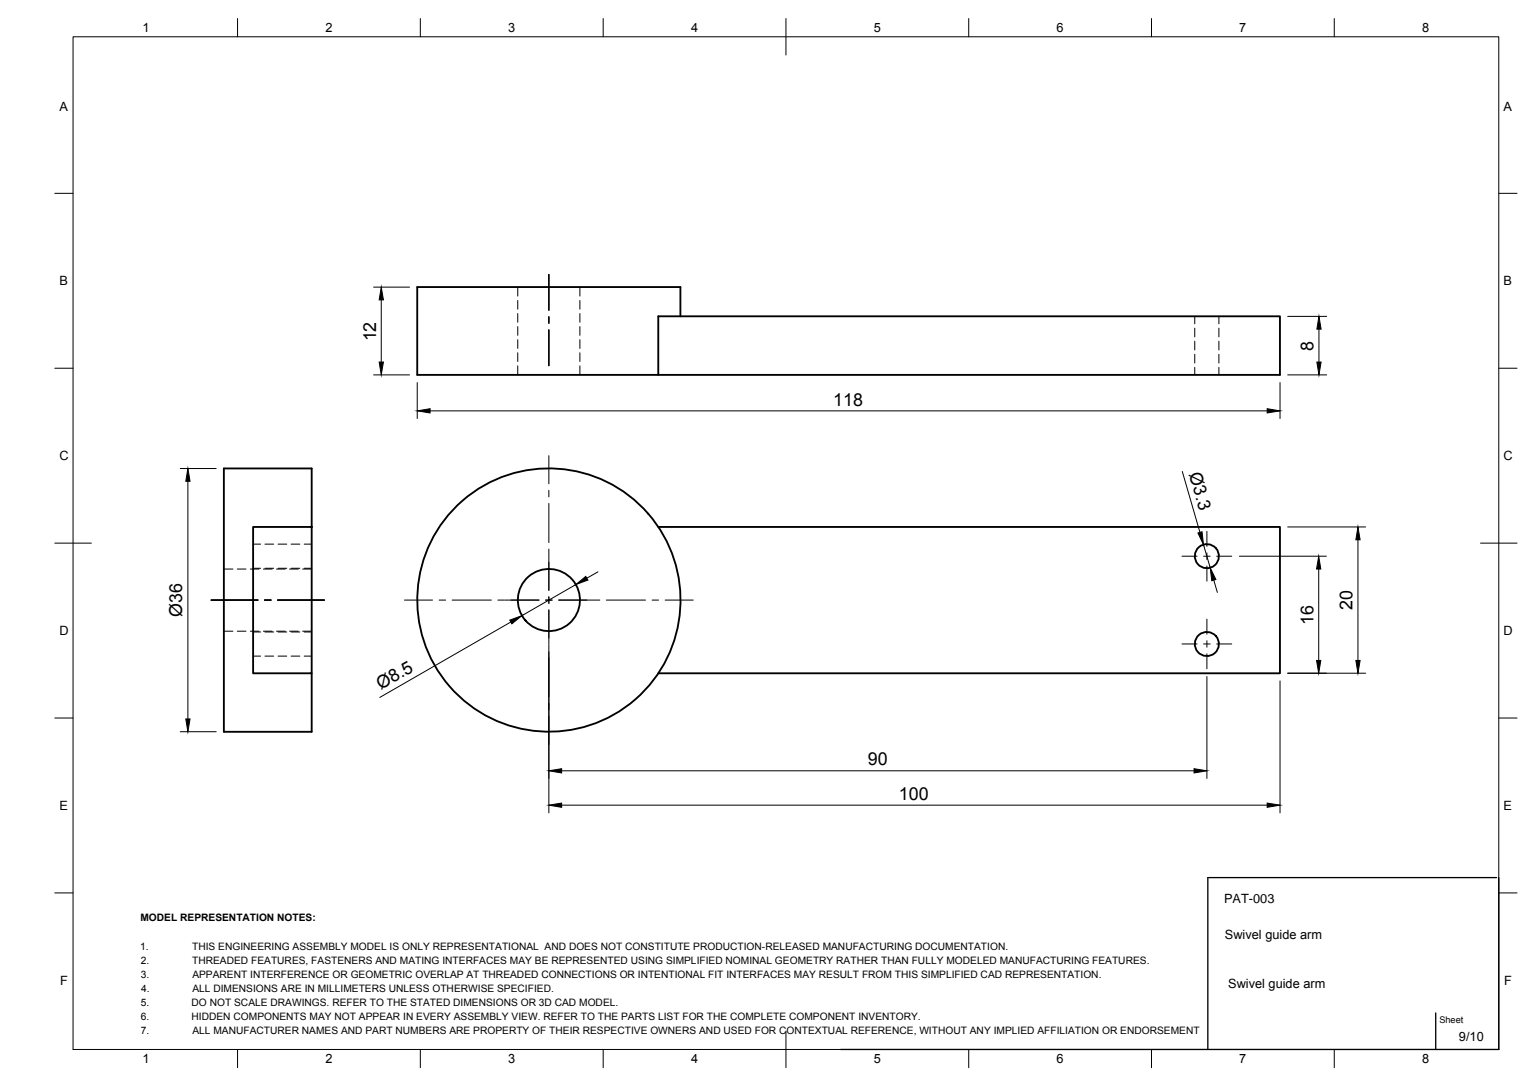
ISO-10303-21;
HEADER;
/* Generated by software containing ST-Developer
 * from STEP Tools, Inc. (www.steptools.com) 
 */

FILE_DESCRIPTION(
/* description */ ('PAT-003'),
/* implementation_level */ '2;1');

FILE_NAME(
/* name */ 'Swivel guide arm.step',
/* time_stamp */ '2026-10-29T15:45:40-07:00',
/* author */ (''),
/* organization */ (''),
/* preprocessor_version */ 'ST-DEVELOPER v20.2',
/* originating_system */ 'Autodesk Translation Framework v15.17.0.0',
/* authorisation */ '');

FILE_SCHEMA (('AUTOMOTIVE_DESIGN { 1 0 10303 214 3 1 1 }'));
ENDSEC;

DATA;
#10=MECHANICAL_DESIGN_GEOMETRIC_PRESENTATION_REPRESENTATION('',(#153),#5761);
#129=SHAPE_REPRESENTATION_RELATIONSHIP('SRR','None',#5824,#141);
#141=ADVANCED_BREP_SHAPE_REPRESENTATION('',(#164),#5755);
#153=STYLED_ITEM('',(#5942),#164);
#164=MANIFOLD_SOLID_BREP('Body1',#3328);
#186=FACE_BOUND('',#659,.T.);
#187=FACE_BOUND('',#660,.T.);
#188=FACE_BOUND('',#661,.T.);
#189=FACE_BOUND('',#666,.T.);
#190=FACE_BOUND('',#667,.T.);
#191=FACE_BOUND('',#671,.T.);
#297=PLANE('',#3633);
#298=PLANE('',#3637);
#299=PLANE('',#3638);
#300=PLANE('',#3639);
#301=PLANE('',#3640);
#302=PLANE('',#3646);
#452=FACE_OUTER_BOUND('',#656,.T.);
#453=FACE_OUTER_BOUND('',#657,.T.);
#454=FACE_OUTER_BOUND('',#658,.T.);
#455=FACE_OUTER_BOUND('',#662,.T.);
#456=FACE_OUTER_BOUND('',#663,.T.);
#457=FACE_OUTER_BOUND('',#664,.T.);
#458=FACE_OUTER_BOUND('',#665,.T.);
#459=FACE_OUTER_BOUND('',#668,.T.);
#460=FACE_OUTER_BOUND('',#669,.T.);
#461=FACE_OUTER_BOUND('',#670,.T.);
#656=EDGE_LOOP('',(#2758,#2759,#2760,#2761));
#657=EDGE_LOOP('',(#2762,#2763,#2764,#2765));
#658=EDGE_LOOP('',(#2766,#2767,#2768,#2769,#2770));
#659=EDGE_LOOP('',(#2771));
#660=EDGE_LOOP('',(#2772));
#661=EDGE_LOOP('',(#2773));
#662=EDGE_LOOP('',(#2774,#2775,#2776,#2777));
#663=EDGE_LOOP('',(#2778,#2779,#2780,#2781));
#664=EDGE_LOOP('',(#2782,#2783,#2784,#2785));
#665=EDGE_LOOP('',(#2786,#2787,#2788,#2789));
#666=EDGE_LOOP('',(#2790));
#667=EDGE_LOOP('',(#2791));
#668=EDGE_LOOP('',(#2792,#2793,#2794,#2795,#2796,#2797,#2798,#2799));
#669=EDGE_LOOP('',(#2800,#2801,#2802,#2803));
#670=EDGE_LOOP('',(#2804));
#671=EDGE_LOOP('',(#2805));
#978=LINE('',#5332,#1300);
#979=LINE('',#5338,#1301);
#980=LINE('',#5347,#1302);
#981=LINE('',#5349,#1303);
#982=LINE('',#5350,#1304);
#983=LINE('',#5355,#1305);
#984=LINE('',#5357,#1306);
#985=LINE('',#5358,#1307);
#986=LINE('',#5361,#1308);
#987=LINE('',#5362,#1309);
#988=LINE('',#5365,#1310);
#989=LINE('',#5366,#1311);
#990=LINE('',#5371,#1312);
#991=LINE('',#5375,#1313);
#1300=VECTOR('',#4335,0.164999999999999);
#1301=VECTOR('',#4342,0.164999999999999);
#1302=VECTOR('',#4351,1.);
#1303=VECTOR('',#4352,1.);
#1304=VECTOR('',#4353,1.);
#1305=VECTOR('',#4358,1.);
#1306=VECTOR('',#4359,1.);
#1307=VECTOR('',#4360,1.);
#1308=VECTOR('',#4363,1.);
#1309=VECTOR('',#4364,1.);
#1310=VECTOR('',#4367,1.);
#1311=VECTOR('',#4368,1.);
#1312=VECTOR('',#4375,1.8);
#1313=VECTOR('',#4380,0.425);
#1432=CIRCLE('',#3628,0.164999999999999);
#1433=CIRCLE('',#3629,0.164999999999999);
#1434=CIRCLE('',#3631,0.164999999999999);
#1435=CIRCLE('',#3632,0.164999999999999);
#1436=CIRCLE('',#3634,1.8);
#1437=CIRCLE('',#3635,1.8);
#1438=CIRCLE('',#3636,0.425);
#1439=CIRCLE('',#3641,1.8);
#1440=CIRCLE('',#3643,1.8);
#1441=CIRCLE('',#3645,0.425);
#1670=VERTEX_POINT('',#5329);
#1671=VERTEX_POINT('',#5331);
#1672=VERTEX_POINT('',#5335);
#1673=VERTEX_POINT('',#5337);
#1674=VERTEX_POINT('',#5341);
#1675=VERTEX_POINT('',#5342);
#1676=VERTEX_POINT('',#5344);
#1677=VERTEX_POINT('',#5346);
#1678=VERTEX_POINT('',#5348);
#1679=VERTEX_POINT('',#5351);
#1680=VERTEX_POINT('',#5354);
#1681=VERTEX_POINT('',#5356);
#1682=VERTEX_POINT('',#5360);
#1683=VERTEX_POINT('',#5364);
#1684=VERTEX_POINT('',#5370);
#1685=VERTEX_POINT('',#5374);
#2050=EDGE_CURVE('',#1670,#1670,#1432,.T.);
#2051=EDGE_CURVE('',#1670,#1671,#978,.T.);
#2052=EDGE_CURVE('',#1671,#1671,#1433,.T.);
#2053=EDGE_CURVE('',#1672,#1672,#1434,.T.);
#2054=EDGE_CURVE('',#1672,#1673,#979,.T.);
#2055=EDGE_CURVE('',#1673,#1673,#1435,.T.);
#2056=EDGE_CURVE('',#1674,#1675,#1436,.T.);
#2057=EDGE_CURVE('',#1675,#1676,#1437,.T.);
#2058=EDGE_CURVE('',#1676,#1677,#980,.T.);
#2059=EDGE_CURVE('',#1677,#1678,#981,.T.);
#2060=EDGE_CURVE('',#1678,#1674,#982,.T.);
#2061=EDGE_CURVE('',#1679,#1679,#1438,.T.);
#2062=EDGE_CURVE('',#1674,#1680,#983,.T.);
#2063=EDGE_CURVE('',#1681,#1678,#984,.T.);
#2064=EDGE_CURVE('',#1681,#1680,#985,.T.);
#2065=EDGE_CURVE('',#1682,#1681,#986,.T.);
#2066=EDGE_CURVE('',#1682,#1677,#987,.T.);
#2067=EDGE_CURVE('',#1683,#1676,#988,.T.);
#2068=EDGE_CURVE('',#1683,#1682,#989,.T.);
#2069=EDGE_CURVE('',#1680,#1683,#1439,.T.);
#2070=EDGE_CURVE('',#1675,#1684,#990,.T.);
#2071=EDGE_CURVE('',#1684,#1684,#1440,.T.);
#2072=EDGE_CURVE('',#1679,#1685,#991,.T.);
#2073=EDGE_CURVE('',#1685,#1685,#1441,.T.);
#2758=ORIENTED_EDGE('',*,*,#2050,.F.);
#2759=ORIENTED_EDGE('',*,*,#2051,.T.);
#2760=ORIENTED_EDGE('',*,*,#2052,.F.);
#2761=ORIENTED_EDGE('',*,*,#2051,.F.);
#2762=ORIENTED_EDGE('',*,*,#2053,.F.);
#2763=ORIENTED_EDGE('',*,*,#2054,.T.);
#2764=ORIENTED_EDGE('',*,*,#2055,.F.);
#2765=ORIENTED_EDGE('',*,*,#2054,.F.);
#2766=ORIENTED_EDGE('',*,*,#2056,.T.);
#2767=ORIENTED_EDGE('',*,*,#2057,.T.);
#2768=ORIENTED_EDGE('',*,*,#2058,.T.);
#2769=ORIENTED_EDGE('',*,*,#2059,.T.);
#2770=ORIENTED_EDGE('',*,*,#2060,.T.);
#2771=ORIENTED_EDGE('',*,*,#2052,.T.);
#2772=ORIENTED_EDGE('',*,*,#2055,.T.);
#2773=ORIENTED_EDGE('',*,*,#2061,.T.);
#2774=ORIENTED_EDGE('',*,*,#2062,.F.);
#2775=ORIENTED_EDGE('',*,*,#2060,.F.);
#2776=ORIENTED_EDGE('',*,*,#2063,.F.);
#2777=ORIENTED_EDGE('',*,*,#2064,.T.);
#2778=ORIENTED_EDGE('',*,*,#2065,.T.);
#2779=ORIENTED_EDGE('',*,*,#2063,.T.);
#2780=ORIENTED_EDGE('',*,*,#2059,.F.);
#2781=ORIENTED_EDGE('',*,*,#2066,.F.);
#2782=ORIENTED_EDGE('',*,*,#2067,.F.);
#2783=ORIENTED_EDGE('',*,*,#2068,.T.);
#2784=ORIENTED_EDGE('',*,*,#2066,.T.);
#2785=ORIENTED_EDGE('',*,*,#2058,.F.);
#2786=ORIENTED_EDGE('',*,*,#2069,.F.);
#2787=ORIENTED_EDGE('',*,*,#2064,.F.);
#2788=ORIENTED_EDGE('',*,*,#2065,.F.);
#2789=ORIENTED_EDGE('',*,*,#2068,.F.);
#2790=ORIENTED_EDGE('',*,*,#2050,.T.);
#2791=ORIENTED_EDGE('',*,*,#2053,.T.);
#2792=ORIENTED_EDGE('',*,*,#2062,.T.);
#2793=ORIENTED_EDGE('',*,*,#2069,.T.);
#2794=ORIENTED_EDGE('',*,*,#2067,.T.);
#2795=ORIENTED_EDGE('',*,*,#2057,.F.);
#2796=ORIENTED_EDGE('',*,*,#2070,.T.);
#2797=ORIENTED_EDGE('',*,*,#2071,.T.);
#2798=ORIENTED_EDGE('',*,*,#2070,.F.);
#2799=ORIENTED_EDGE('',*,*,#2056,.F.);
#2800=ORIENTED_EDGE('',*,*,#2061,.F.);
#2801=ORIENTED_EDGE('',*,*,#2072,.T.);
#2802=ORIENTED_EDGE('',*,*,#2073,.T.);
#2803=ORIENTED_EDGE('',*,*,#2072,.F.);
#2804=ORIENTED_EDGE('',*,*,#2071,.F.);
#2805=ORIENTED_EDGE('',*,*,#2073,.F.);
#3108=CYLINDRICAL_SURFACE('',#3627,0.164999999999999);
#3109=CYLINDRICAL_SURFACE('',#3630,0.164999999999999);
#3110=CYLINDRICAL_SURFACE('',#3642,1.8);
#3111=CYLINDRICAL_SURFACE('',#3644,0.425);
#3245=ADVANCED_FACE('',(#452),#3108,.F.);
#3246=ADVANCED_FACE('',(#453),#3109,.F.);
#3247=ADVANCED_FACE('',(#454,#186,#187,#188),#297,.T.);
#3248=ADVANCED_FACE('',(#455),#298,.T.);
#3249=ADVANCED_FACE('',(#456),#299,.T.);
#3250=ADVANCED_FACE('',(#457),#300,.T.);
#3251=ADVANCED_FACE('',(#458,#189,#190),#301,.F.);
#3252=ADVANCED_FACE('',(#459),#3110,.T.);
#3253=ADVANCED_FACE('',(#460),#3111,.F.);
#3254=ADVANCED_FACE('',(#461,#191),#302,.F.);
#3328=CLOSED_SHELL('',(#3245,#3246,#3247,#3248,#3249,#3250,#3251,#3252,
#3253,#3254));
#3626=AXIS2_PLACEMENT_3D('',#5327,#4329,#4330);
#3627=AXIS2_PLACEMENT_3D('',#5328,#4331,#4332);
#3628=AXIS2_PLACEMENT_3D('',#5330,#4333,#4334);
#3629=AXIS2_PLACEMENT_3D('',#5333,#4336,#4337);
#3630=AXIS2_PLACEMENT_3D('',#5334,#4338,#4339);
#3631=AXIS2_PLACEMENT_3D('',#5336,#4340,#4341);
#3632=AXIS2_PLACEMENT_3D('',#5339,#4343,#4344);
#3633=AXIS2_PLACEMENT_3D('',#5340,#4345,#4346);
#3634=AXIS2_PLACEMENT_3D('',#5343,#4347,#4348);
#3635=AXIS2_PLACEMENT_3D('',#5345,#4349,#4350);
#3636=AXIS2_PLACEMENT_3D('',#5352,#4354,#4355);
#3637=AXIS2_PLACEMENT_3D('',#5353,#4356,#4357);
#3638=AXIS2_PLACEMENT_3D('',#5359,#4361,#4362);
#3639=AXIS2_PLACEMENT_3D('',#5363,#4365,#4366);
#3640=AXIS2_PLACEMENT_3D('',#5367,#4369,#4370);
#3641=AXIS2_PLACEMENT_3D('',#5368,#4371,#4372);
#3642=AXIS2_PLACEMENT_3D('',#5369,#4373,#4374);
#3643=AXIS2_PLACEMENT_3D('',#5372,#4376,#4377);
#3644=AXIS2_PLACEMENT_3D('',#5373,#4378,#4379);
#3645=AXIS2_PLACEMENT_3D('',#5376,#4381,#4382);
#3646=AXIS2_PLACEMENT_3D('',#5377,#4383,#4384);
#4329=DIRECTION('axis',(0.,0.,1.));
#4330=DIRECTION('refdir',(1.,0.,0.));
#4331=DIRECTION('center_axis',(0.,0.,1.));
#4332=DIRECTION('ref_axis',(1.,0.,0.));
#4333=DIRECTION('center_axis',(0.,0.,1.));
#4334=DIRECTION('ref_axis',(1.,0.,0.));
#4335=DIRECTION('',(0.,0.,1.));
#4336=DIRECTION('center_axis',(0.,0.,-1.));
#4337=DIRECTION('ref_axis',(1.,0.,0.));
#4338=DIRECTION('center_axis',(0.,0.,1.));
#4339=DIRECTION('ref_axis',(1.,0.,0.));
#4340=DIRECTION('center_axis',(0.,0.,1.));
#4341=DIRECTION('ref_axis',(1.,0.,0.));
#4342=DIRECTION('',(0.,0.,1.));
#4343=DIRECTION('center_axis',(0.,0.,-1.));
#4344=DIRECTION('ref_axis',(1.,0.,0.));
#4345=DIRECTION('center_axis',(0.,0.,1.));
#4346=DIRECTION('ref_axis',(1.,0.,0.));
#4347=DIRECTION('center_axis',(0.,0.,1.));
#4348=DIRECTION('ref_axis',(1.,0.,0.));
#4349=DIRECTION('center_axis',(0.,0.,1.));
#4350=DIRECTION('ref_axis',(1.,0.,0.));
#4351=DIRECTION('',(1.,0.,0.));
#4352=DIRECTION('',(0.,1.,0.));
#4353=DIRECTION('',(-1.,0.,0.));
#4354=DIRECTION('center_axis',(0.,0.,-1.));
#4355=DIRECTION('ref_axis',(1.,0.,0.));
#4356=DIRECTION('center_axis',(0.,1.,0.));
#4357=DIRECTION('ref_axis',(-1.,0.,0.));
#4358=DIRECTION('',(0.,0.,-1.));
#4359=DIRECTION('',(0.,0.,1.));
#4360=DIRECTION('',(-1.,0.,0.));
#4361=DIRECTION('center_axis',(1.,0.,0.));
#4362=DIRECTION('ref_axis',(0.,1.,0.));
#4363=DIRECTION('',(0.,1.,0.));
#4364=DIRECTION('',(0.,0.,1.));
#4365=DIRECTION('center_axis',(0.,-1.,0.));
#4366=DIRECTION('ref_axis',(1.,0.,0.));
#4367=DIRECTION('',(0.,0.,1.));
#4368=DIRECTION('',(1.,0.,0.));
#4369=DIRECTION('center_axis',(0.,0.,1.));
#4370=DIRECTION('ref_axis',(1.,0.,0.));
#4371=DIRECTION('center_axis',(0.,0.,-1.));
#4372=DIRECTION('ref_axis',(1.,0.,0.));
#4373=DIRECTION('center_axis',(0.,0.,1.));
#4374=DIRECTION('ref_axis',(1.,0.,0.));
#4375=DIRECTION('',(0.,0.,-1.));
#4376=DIRECTION('center_axis',(0.,0.,1.));
#4377=DIRECTION('ref_axis',(1.,0.,0.));
#4378=DIRECTION('center_axis',(0.,0.,1.));
#4379=DIRECTION('ref_axis',(1.,0.,0.));
#4380=DIRECTION('',(0.,0.,-1.));
#4381=DIRECTION('center_axis',(0.,0.,-1.));
#4382=DIRECTION('ref_axis',(1.,0.,0.));
#4383=DIRECTION('center_axis',(0.,0.,1.));
#4384=DIRECTION('ref_axis',(1.,0.,0.));
#5327=CARTESIAN_POINT('',(0.,0.,0.));
#5328=CARTESIAN_POINT('Origin',(14.,-0.6,4.7));
#5329=CARTESIAN_POINT('',(13.835,-0.6,4.8));
#5330=CARTESIAN_POINT('Origin',(14.,-0.6,4.8));
#5331=CARTESIAN_POINT('',(13.835,-0.6,5.6));
#5332=CARTESIAN_POINT('',(13.835,-0.6,4.7));
#5333=CARTESIAN_POINT('Origin',(14.,-0.6,5.6));
#5334=CARTESIAN_POINT('Origin',(14.,0.6,4.7));
#5335=CARTESIAN_POINT('',(13.835,0.6,4.8));
#5336=CARTESIAN_POINT('Origin',(14.,0.6,4.8));
#5337=CARTESIAN_POINT('',(13.835,0.6,5.6));
#5338=CARTESIAN_POINT('',(13.835,0.6,4.7));
#5339=CARTESIAN_POINT('Origin',(14.,0.6,5.6));
#5340=CARTESIAN_POINT('Origin',(5.,0.,5.6));
#5341=CARTESIAN_POINT('',(6.49666295470958,1.,5.6));
#5342=CARTESIAN_POINT('',(3.2,-2.20436423846524E-16,5.6));
#5343=CARTESIAN_POINT('Origin',(5.,0.,5.6));
#5344=CARTESIAN_POINT('',(6.49666295470958,-1.,5.6));
#5345=CARTESIAN_POINT('Origin',(5.,0.,5.6));
#5346=CARTESIAN_POINT('',(15.,-1.,5.6));
#5347=CARTESIAN_POINT('',(5.,-1.,5.6));
#5348=CARTESIAN_POINT('',(15.,1.,5.6));
#5349=CARTESIAN_POINT('',(15.,-1.,5.6));
#5350=CARTESIAN_POINT('',(15.,1.,5.6));
#5351=CARTESIAN_POINT('',(4.575,-5.20474889637625E-17,5.6));
#5352=CARTESIAN_POINT('Origin',(5.,0.,5.6));
#5353=CARTESIAN_POINT('Origin',(15.,1.,4.8));
#5354=CARTESIAN_POINT('',(6.49666295470958,1.,4.8));
#5355=CARTESIAN_POINT('',(6.49666295470958,1.,4.4));
#5356=CARTESIAN_POINT('',(15.,1.,4.8));
#5357=CARTESIAN_POINT('',(15.,1.,4.8));
#5358=CARTESIAN_POINT('',(15.,1.,4.8));
#5359=CARTESIAN_POINT('Origin',(15.,-1.,4.8));
#5360=CARTESIAN_POINT('',(15.,-1.,4.8));
#5361=CARTESIAN_POINT('',(15.,-1.,4.8));
#5362=CARTESIAN_POINT('',(15.,-1.,4.8));
#5363=CARTESIAN_POINT('Origin',(5.,-1.,4.8));
#5364=CARTESIAN_POINT('',(6.49666295470958,-1.,4.8));
#5365=CARTESIAN_POINT('',(6.49666295470958,-1.,4.4));
#5366=CARTESIAN_POINT('',(5.,-1.,4.8));
#5367=CARTESIAN_POINT('Origin',(10.,0.,4.8));
#5368=CARTESIAN_POINT('Origin',(5.,0.,4.8));
#5369=CARTESIAN_POINT('Origin',(5.,0.,4.4));
#5370=CARTESIAN_POINT('',(3.2,-2.20436423846524E-16,4.4));
#5371=CARTESIAN_POINT('',(3.2,-2.20436423846524E-16,4.4));
#5372=CARTESIAN_POINT('Origin',(5.,0.,4.4));
#5373=CARTESIAN_POINT('Origin',(5.,0.,4.4));
#5374=CARTESIAN_POINT('',(4.575,-5.20474889637625E-17,4.4));
#5375=CARTESIAN_POINT('',(4.575,-5.20474889637625E-17,4.4));
#5376=CARTESIAN_POINT('Origin',(5.,0.,4.4));
#5377=CARTESIAN_POINT('Origin',(5.,0.,4.4));
#5739=UNCERTAINTY_MEASURE_WITH_UNIT(LENGTH_MEASURE(0.001),#5762,
'DISTANCE_ACCURACY_VALUE',
'Maximum model space distance between geometric entities at asserted c
onnectivities');
#5745=UNCERTAINTY_MEASURE_WITH_UNIT(LENGTH_MEASURE(0.001),#5762,
'DISTANCE_ACCURACY_VALUE',
'Maximum model space distance between geometric entities at asserted c
onnectivities');
#5755=(
GEOMETRIC_REPRESENTATION_CONTEXT(3)
GLOBAL_UNCERTAINTY_ASSIGNED_CONTEXT((#5739))
GLOBAL_UNIT_ASSIGNED_CONTEXT((#5762,#5764,#5765))
REPRESENTATION_CONTEXT('','3D')
);
#5761=(
GEOMETRIC_REPRESENTATION_CONTEXT(3)
GLOBAL_UNCERTAINTY_ASSIGNED_CONTEXT((#5745))
GLOBAL_UNIT_ASSIGNED_CONTEXT((#5762,#5764,#5765))
REPRESENTATION_CONTEXT('','3D')
);
#5762=(
LENGTH_UNIT()
NAMED_UNIT(*)
SI_UNIT(.CENTI.,.METRE.)
);
#5764=(
NAMED_UNIT(*)
PLANE_ANGLE_UNIT()
SI_UNIT($,.RADIAN.)
);
#5765=(
NAMED_UNIT(*)
SI_UNIT($,.STERADIAN.)
SOLID_ANGLE_UNIT()
);
#5775=SHAPE_DEFINITION_REPRESENTATION(#5790,#5824);
#5790=PRODUCT_DEFINITION_SHAPE('',$,#5840);
#5824=SHAPE_REPRESENTATION('',(#3626),#5755);
#5830=PRODUCT_DEFINITION_CONTEXT('part definition',#5877,'design');
#5840=PRODUCT_DEFINITION('Swivel guide arm','Swivel guide arm',#5855,#5830);
#5855=PRODUCT_DEFINITION_FORMATION('',$,#5888);
#5877=APPLICATION_CONTEXT(
'Core Data for Automotive Mechanical Design Process');
#5878=PRODUCT_CONTEXT('part definition',#5877,'mechanical');
#5888=PRODUCT('Swivel guide arm','Swivel guide arm','Swivel guide arm',
(#5878));
#5936=COLOUR_RGB('Sky Blue',0.24,0.69,0.87);
#5937=FILL_AREA_STYLE_COLOUR('',#5936);
#5938=FILL_AREA_STYLE('',(#5937));
#5939=SURFACE_STYLE_FILL_AREA(#5938);
#5940=SURFACE_SIDE_STYLE('',(#5939));
#5941=SURFACE_STYLE_USAGE(.BOTH.,#5940);
#5942=PRESENTATION_STYLE_ASSIGNMENT((#5941));
ENDSEC;
END-ISO-10303-21;
